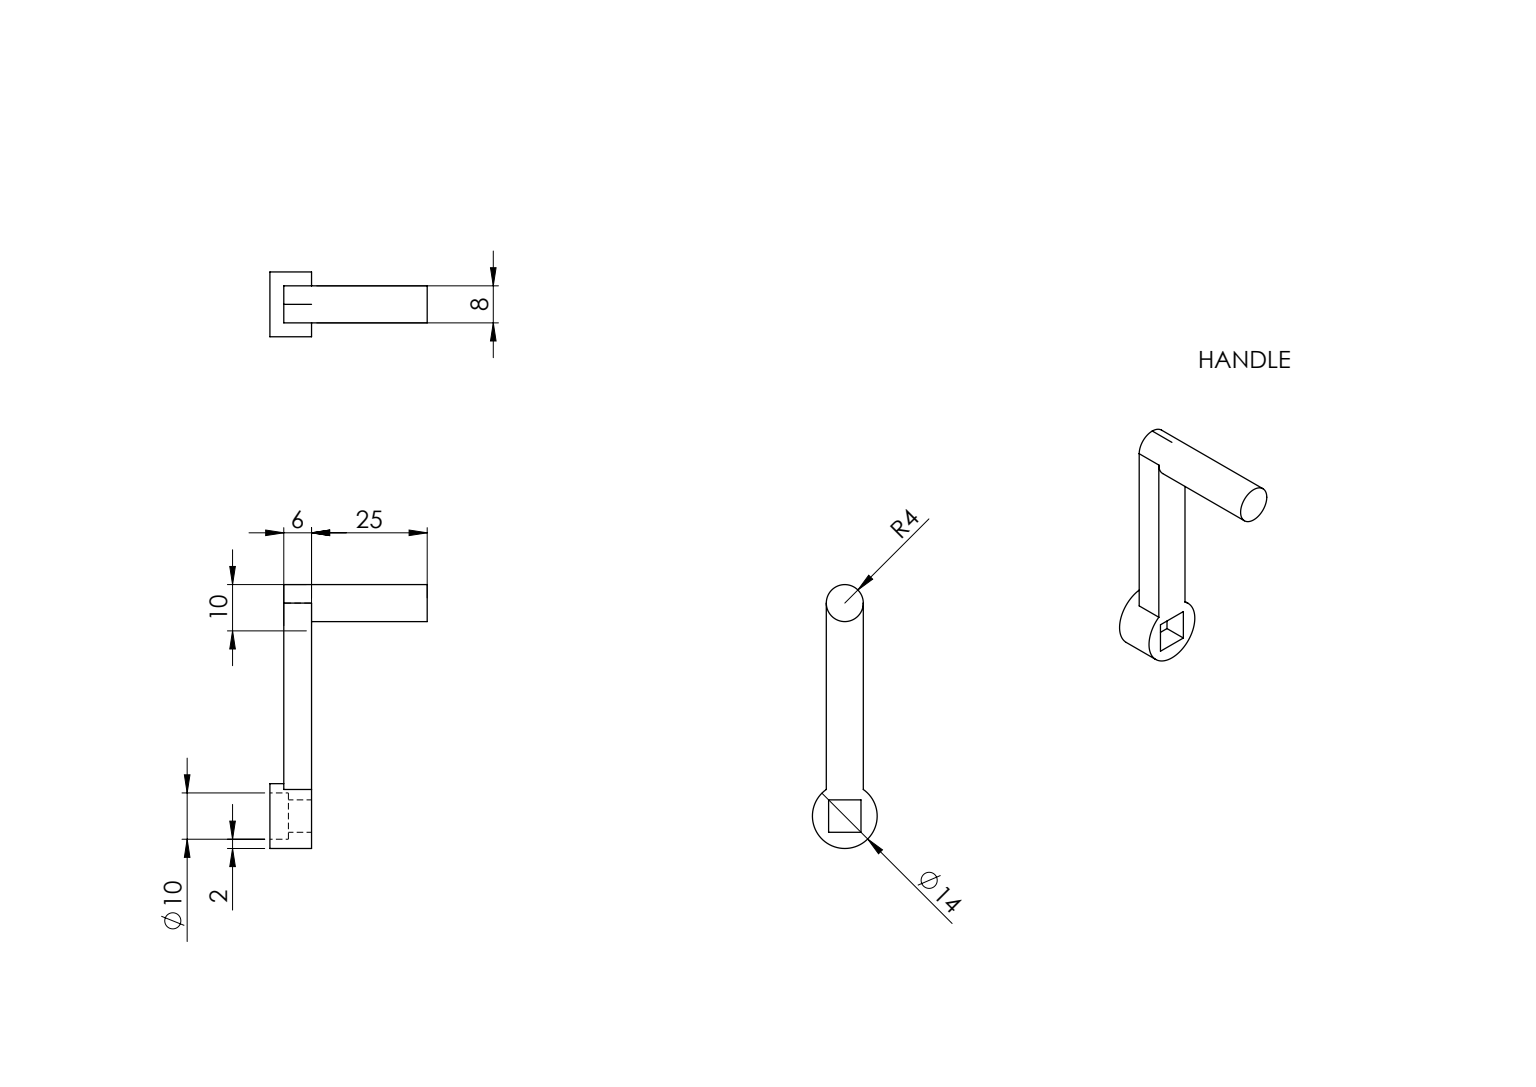
ISO-10303-21;
HEADER;
FILE_DESCRIPTION (('STEP AP214'),
    '1' );
FILE_NAME ('handle.step',
    '2026-10-27T08:02:39',
    ( '' ),
    ( '' ),
    'SwSTEP 2.0',
    'SolidWorks 2026',
    '' );
FILE_SCHEMA (( 'AUTOMOTIVE_DESIGN' ));
ENDSEC;

DATA;
#27=EDGE_LOOP ( 'NONE', ( #3716, #7736, #9091, #8420 ) ) ;
#71=( LENGTH_UNIT ( ) NAMED_UNIT ( * ) SI_UNIT ( .MILLI., .METRE. ) );
#105=LINE ( 'NONE', #3865, #7814 ) ;
#108=EDGE_CURVE ( 'NONE', #8484, #432, #5151, .T. ) ;
#117=DIRECTION ( 'NONE',  ( 0.000000000000000000, 0.000000000000000000, 1.000000000000000000 ) ) ;
#124=DIRECTION ( 'NONE',  ( 0.000000000000000000, 0.000000000000000000, 1.000000000000000000 ) ) ;
#170=VERTEX_POINT ( 'NONE', #7231 ) ;
#212=CARTESIAN_POINT ( 'NONE',  ( 0.000000000000000000, 0.000000000000000000, 0.000000000000000000 ) ) ;
#216=AXIS2_PLACEMENT_3D ( 'NONE', #497, #4306, #3323 ) ;
#249=FACE_OUTER_BOUND ( 'NONE', #9270, .T. ) ;
#265=EDGE_CURVE ( 'NONE', #8484, #2318, #5290, .T. ) ;
#277=CARTESIAN_POINT ( 'NONE',  ( 0.000000000000000000, 46.00000000000001421, -41.99999999999999289 ) ) ;
#311=EDGE_LOOP ( 'NONE', ( #6611, #4902, #12095, #9968, #4063 ) ) ;
#312=LINE ( 'NONE', #2306, #8963 ) ;
#316=CARTESIAN_POINT ( 'NONE',  ( 45.00000000000001421, 50.00000000000000711, -46.00000000000000000 ) ) ;
#333=CARTESIAN_POINT ( 'NONE',  ( 65.79898987322334847, -9.445087446769608850E-17, -41.99999999999998579 ) ) ;
#361=VECTOR ( 'NONE', #839, 1000.000000000000000 ) ;
#362=CARTESIAN_POINT ( 'NONE',  ( 42.00000000000000000, 1.908195823574506293E-17, -41.99999999999998579 ) ) ;
#378=ORIENTED_EDGE ( 'NONE', *, *, #265, .F. ) ;
#413=LINE ( 'NONE', #4060, #11148 ) ;
#432=VERTEX_POINT ( 'NONE', #10181 ) ;
#443=DIRECTION ( 'NONE',  ( 0.000000000000000000, 0.000000000000000000, 1.000000000000000000 ) ) ;
#488=ORIENTED_EDGE ( 'NONE', *, *, #5345, .F. ) ;
#495=EDGE_CURVE ( 'NONE', #1234, #3139, #11361, .T. ) ;
#497=CARTESIAN_POINT ( 'NONE',  ( 45.00000000000001421, 4.770489558936308102E-18, -41.99999999999998579 ) ) ;
#677=CIRCLE ( 'NONE', #7465, 5.000000000000004441 ) ;
#683=AXIS2_PLACEMENT_3D ( 'NONE', #333, #4146, #1473 ) ;
#699=CIRCLE ( 'NONE', #3309, 7.000000000000006217 ) ;
#730=DIRECTION ( 'NONE',  ( 1.000000000000000000, 0.000000000000000000, 0.000000000000000000 ) ) ;
#756=CARTESIAN_POINT ( 'NONE',  ( 65.79898987322334847, -9.445087446769608850E-17, -41.99999999999998579 ) ) ;
#758=AXIS2_PLACEMENT_3D ( 'NONE', #5741, #8694, #117 ) ;
#761=ORIENTED_EDGE ( 'NONE', *, *, #8385, .F. ) ;
#811=VERTEX_POINT ( 'NONE', #6939 ) ;
#839=DIRECTION ( 'NONE',  ( 1.000000000000000000, -4.770489558936236458E-18, 6.855277276495154548E-34 ) ) ;
#858=LINE ( 'NONE', #11064, #11986 ) ;
#871=EDGE_CURVE ( 'NONE', #3139, #7019, #10116, .T. ) ;
#884=EDGE_CURVE ( 'NONE', #5539, #7662, #4798, .T. ) ;
#892=EDGE_LOOP ( 'NONE', ( #2724, #5114, #7799, #6342 ) ) ;
#905=DIRECTION ( 'NONE',  ( -1.000000000000000000, -0.000000000000000000, -0.000000000000000000 ) ) ;
#936=( NAMED_UNIT ( * ) SI_UNIT ( $, .STERADIAN. ) SOLID_ANGLE_UNIT ( ) );
#953=EDGE_CURVE ( 'NONE', #8701, #7793, #8813, .T. ) ;
#960=ORIENTED_EDGE ( 'NONE', *, *, #7258, .T. ) ;
#968=EDGE_CURVE ( 'NONE', #2318, #8881, #10351, .T. ) ;
#999=SURFACE_STYLE_FILL_AREA ( #8572 ) ;
#1040=AXIS2_PLACEMENT_3D ( 'NONE', #277, #8722, #1092 ) ;
#1076=EDGE_CURVE ( 'NONE', #3524, #10474, #105, .T. ) ;
#1092=DIRECTION ( 'NONE',  ( 0.000000000000000000, 0.000000000000000000, -1.000000000000000000 ) ) ;
#1094=VERTEX_POINT ( 'NONE', #10483 ) ;
#1110=DIRECTION ( 'NONE',  ( 1.000000000000000000, 0.000000000000000000, 0.000000000000000000 ) ) ;
#1174=EDGE_CURVE ( 'NONE', #7662, #5539, #10599, .T. ) ;
#1176=DIRECTION ( 'NONE',  ( 1.000000000000000000, 0.000000000000000000, 0.000000000000000000 ) ) ;
#1223=ORIENTED_EDGE ( 'NONE', *, *, #871, .T. ) ;
#1234=VERTEX_POINT ( 'NONE', #9922 ) ;
#1307=DIRECTION ( 'NONE',  ( 1.000000000000000000, -4.770489558936236458E-18, 6.855277276495153692E-34 ) ) ;
#1321=PLANE ( 'NONE',  #8288 ) ;
#1368=CYLINDRICAL_SURFACE ( 'NONE', #11978, 7.000000000000004441 ) ;
#1414=ADVANCED_FACE ( 'NONE', ( #3479 ), #2525, .T. ) ;
#1418=ADVANCED_FACE ( 'NONE', ( #9115 ), #8166, .F. ) ;
#1444=AXIS2_PLACEMENT_3D ( 'NONE', #316, #443, #11744 ) ;
#1473=DIRECTION ( 'NONE',  ( 0.000000000000000000, -1.000000000000000000, 0.000000000000000000 ) ) ;
#1497=EDGE_CURVE ( 'NONE', #8881, #432, #11394, .T. ) ;
#1509=DIRECTION ( 'NONE',  ( -1.000000000000000000, 0.000000000000000000, -0.000000000000000000 ) ) ;
#1515=ORIENTED_EDGE ( 'NONE', *, *, #7216, .T. ) ;
#1552=ADVANCED_FACE ( 'NONE', ( #6730, #2960 ), #4771, .F. ) ;
#1573=DIRECTION ( 'NONE',  ( 0.000000000000000000, 1.000000000000000000, 0.000000000000000000 ) ) ;
#1576=DIRECTION ( 'NONE',  ( 0.000000000000000000, 0.000000000000000000, -1.000000000000000000 ) ) ;
#1590=CARTESIAN_POINT ( 'NONE',  ( 45.00000000000001421, 50.00000000000000711, -38.00000000000000000 ) ) ;
#1622=AXIS2_PLACEMENT_3D ( 'NONE', #4950, #7720, #6772 ) ;
#1645=DIRECTION ( 'NONE',  ( 1.000000000000000000, -0.000000000000000000, 0.000000000000000000 ) ) ;
#1652=FACE_OUTER_BOUND ( 'NONE', #12014, .T. ) ;
#1663=DIRECTION ( 'NONE',  ( 0.000000000000000000, -1.000000000000000000, 0.000000000000000000 ) ) ;
#1696=DIRECTION ( 'NONE',  ( 0.000000000000000000, 0.000000000000000000, 1.000000000000000000 ) ) ;
#1770=AXIS2_PLACEMENT_3D ( 'NONE', #7783, #8594, #8665 ) ;
#1784=SHAPE_DEFINITION_REPRESENTATION ( #10198, #8426 ) ;
#1801=EDGE_CURVE ( 'NONE', #10474, #1992, #3521, .T. ) ;
#1808=VECTOR ( 'NONE', #1573, 1000.000000000000000 ) ;
#1887=( GEOMETRIC_REPRESENTATION_CONTEXT ( 3 ) GLOBAL_UNCERTAINTY_ASSIGNED_CONTEXT ( ( #4523 ) ) GLOBAL_UNIT_ASSIGNED_CONTEXT ( ( #4965, #6678, #5723 ) ) REPRESENTATION_CONTEXT ( 'NONE', 'WORKASPACE' ) );
#1905=VERTEX_POINT ( 'NONE', #4756 ) ;
#1931=CARTESIAN_POINT ( 'NONE',  ( 45.00000000000001421, 46.00000000000001421, -38.00000000000000000 ) ) ;
#1944=SURFACE_STYLE_USAGE ( .BOTH. , #2886 ) ;
#1992=VERTEX_POINT ( 'NONE', #2752 ) ;
#2006=CARTESIAN_POINT ( 'NONE',  ( 76.00000000000000000, 46.00000000000001421, -41.99999999999999289 ) ) ;
#2103=DIRECTION ( 'NONE',  ( -0.000000000000000000, -1.000000000000000000, -0.000000000000000000 ) ) ;
#2106=DIRECTION ( 'NONE',  ( 0.000000000000000000, 0.000000000000000000, -1.000000000000000000 ) ) ;
#2125=( NAMED_UNIT ( * ) PLANE_ANGLE_UNIT ( ) SI_UNIT ( $, .RADIAN. ) );
#2130=DIRECTION ( 'NONE',  ( -1.000000000000000000, 0.000000000000000000, -0.000000000000000000 ) ) ;
#2145=FACE_OUTER_BOUND ( 'NONE', #3394, .T. ) ;
#2163=AXIS2_PLACEMENT_3D ( 'NONE', #7632, #7560, #12296 ) ;
#2184=DIRECTION ( 'NONE',  ( 4.770489558936236458E-18, 1.000000000000000000, 0.000000000000000000 ) ) ;
#2220=ORIENTED_EDGE ( 'NONE', *, *, #9403, .F. ) ;
#2253=EDGE_CURVE ( 'NONE', #1094, #8881, #10596, .T. ) ;
#2293=ORIENTED_EDGE ( 'NONE', *, *, #11296, .T. ) ;
#2306=CARTESIAN_POINT ( 'NONE',  ( 45.00000000000001421, 46.00000000000001421, -46.00000000000000000 ) ) ;
#2318=VERTEX_POINT ( 'NONE', #1931 ) ;
#2319=DIRECTION ( 'NONE',  ( 0.000000000000000000, -1.000000000000000000, 0.000000000000000000 ) ) ;
#2333=EDGE_CURVE ( 'NONE', #8484, #8701, #3056, .T. ) ;
#2385=DIRECTION ( 'NONE',  ( -1.000000000000000000, -0.000000000000000000, -0.000000000000000000 ) ) ;
#2442=ORIENTED_EDGE ( 'NONE', *, *, #9009, .T. ) ;
#2505=EDGE_CURVE ( 'NONE', #1094, #7890, #11958, .T. ) ;
#2508=CARTESIAN_POINT ( 'NONE',  ( 51.00000000000000000, 1.444447458290426890E-31, -41.99999999999998579 ) ) ;
#2525=CYLINDRICAL_SURFACE ( 'NONE', #10013, 7.000000000000004441 ) ;
#2530=ORIENTED_EDGE ( 'NONE', *, *, #6325, .F. ) ;
#2555=CARTESIAN_POINT ( 'NONE',  ( 51.00000000000000000, 5.744562646538031281, -46.00000000000000000 ) ) ;
#2576=EDGE_LOOP ( 'NONE', ( #5137, #9790, #5069, #9510 ) ) ;
#2579=VECTOR ( 'NONE', #6955, 1000.000000000000000 ) ;
#2584=VECTOR ( 'NONE', #5375, 1000.000000000000000 ) ;
#2586=DIRECTION ( 'NONE',  ( 0.000000000000000000, 0.000000000000000000, -1.000000000000000000 ) ) ;
#2603=EDGE_LOOP ( 'NONE', ( #8336, #4066 ) ) ;
#2630=LINE ( 'NONE', #8207, #11415 ) ;
#2671=DIRECTION ( 'NONE',  ( 0.000000000000000000, 0.000000000000000000, -1.000000000000000000 ) ) ;
#2683=PLANE ( 'NONE',  #7968 ) ;
#2694=DIRECTION ( 'NONE',  ( 0.000000000000000000, -1.000000000000000000, 0.000000000000000000 ) ) ;
#2702=ORIENTED_EDGE ( 'NONE', *, *, #953, .F. ) ;
#2724=ORIENTED_EDGE ( 'NONE', *, *, #5874, .F. ) ;
#2752=CARTESIAN_POINT ( 'NONE',  ( 46.00000000000000000, 3.500000000000001332, -45.49999999999998579 ) ) ;
#2762=UNCERTAINTY_MEASURE_WITH_UNIT (LENGTH_MEASURE( 1.000000000000000082E-05 ), #8513, 'distance_accuracy_value', 'NONE');
#2861=ORIENTED_EDGE ( 'NONE', *, *, #7930, .T. ) ;
#2886=SURFACE_SIDE_STYLE ('',( #999 ) ) ;
#2960=FACE_OUTER_BOUND ( 'NONE', #5300, .T. ) ;
#2985=VECTOR ( 'NONE', #12159, 1000.000000000000000 ) ;
#3029=AXIS2_PLACEMENT_3D ( 'NONE', #1590, #2586, #11956 ) ;
#3056=LINE ( 'NONE', #11666, #5020 ) ;
#3059=ADVANCED_FACE ( 'NONE', ( #9861 ), #11652, .T. ) ;
#3121=ADVANCED_FACE ( 'NONE', ( #11137 ), #3649, .F. ) ;
#3136=( NAMED_UNIT ( * ) SI_UNIT ( $, .STERADIAN. ) SOLID_ANGLE_UNIT ( ) );
#3139=VERTEX_POINT ( 'NONE', #12124 ) ;
#3158=DIRECTION ( 'NONE',  ( -0.000000000000000000, 1.000000000000000000, 0.000000000000000000 ) ) ;
#3165=ORIENTED_EDGE ( 'NONE', *, *, #8385, .T. ) ;
#3177=CARTESIAN_POINT ( 'NONE',  ( 51.00000000000000000, 3.500000000000001332, -38.49999999999998579 ) ) ;
#3185=VECTOR ( 'NONE', #11275, 1000.000000000000000 ) ;
#3212=DIRECTION ( 'NONE',  ( 0.000000000000000000, -0.000000000000000000, -1.000000000000000000 ) ) ;
#3309=AXIS2_PLACEMENT_3D ( 'NONE', #2508, #6330, #1696 ) ;
#3323=DIRECTION ( 'NONE',  ( 0.000000000000000000, 2.664535259100374514E-15, 1.000000000000000000 ) ) ;
#3344=ORIENTED_EDGE ( 'NONE', *, *, #6728, .F. ) ;
#3349=CARTESIAN_POINT ( 'NONE',  ( 65.79898987322334847, 7.000000000000004441, -41.99999999999998579 ) ) ;
#3394=EDGE_LOOP ( 'NONE', ( #10298, #8483, #1515, #2702 ) ) ;
#3408=DIRECTION ( 'NONE',  ( -1.000000000000000000, 4.770489558936236458E-18, -6.855277276495154548E-34 ) ) ;
#3416=ADVANCED_FACE ( 'NONE', ( #9894 ), #5953, .F. ) ;
#3423=AXIS2_PLACEMENT_3D ( 'NONE', #7291, #1110, #4922 ) ;
#3432=ORIENTED_EDGE ( 'NONE', *, *, #11724, .T. ) ;
#3451=ORIENTED_EDGE ( 'NONE', *, *, #2333, .T. ) ;
#3452=FACE_OUTER_BOUND ( 'NONE', #892, .T. ) ;
#3479=FACE_OUTER_BOUND ( 'NONE', #9340, .T. ) ;
#3482=ORIENTED_EDGE ( 'NONE', *, *, #6191, .T. ) ;
#3499=AXIS2_PLACEMENT_3D ( 'NONE', #362, #1307, #2184 ) ;
#3521=LINE ( 'NONE', #4324, #10151 ) ;
#3524=VERTEX_POINT ( 'NONE', #6903 ) ;
#3526=DIRECTION ( 'NONE',  ( 0.000000000000000000, 0.000000000000000000, 1.000000000000000000 ) ) ;
#3527=VERTEX_POINT ( 'NONE', #10704 ) ;
#3538=ORIENTED_EDGE ( 'NONE', *, *, #5874, .T. ) ;
#3545=DIRECTION ( 'NONE',  ( -1.000000000000000000, 4.770489558936236458E-18, -6.855277276495154548E-34 ) ) ;
#3570=ORIENTED_EDGE ( 'NONE', *, *, #8614, .F. ) ;
#3586=DIRECTION ( 'NONE',  ( -1.000000000000000000, 0.000000000000000000, 0.000000000000000000 ) ) ;
#3588=ORIENTED_EDGE ( 'NONE', *, *, #265, .T. ) ;
#3632=ORIENTED_EDGE ( 'NONE', *, *, #953, .T. ) ;
#3649=PLANE ( 'NONE',  #7440 ) ;
#3673=DIRECTION ( 'NONE',  ( -1.000000000000000000, 4.770489558936236458E-18, -6.855277276495154548E-34 ) ) ;
#3678=CARTESIAN_POINT ( 'NONE',  ( 76.00000000000000000, 46.00000000000001421, -41.99999999999999289 ) ) ;
#3716=ORIENTED_EDGE ( 'NONE', *, *, #1076, .F. ) ;
#3819=FILL_AREA_STYLE_COLOUR ( '', #6637 ) ;
#3865=CARTESIAN_POINT ( 'NONE',  ( 51.00000000000000000, 3.500000000000001332, -45.49999999999998579 ) ) ;
#3934=APPLICATION_CONTEXT ( 'automotive_design' ) ;
#3941=CARTESIAN_POINT ( 'NONE',  ( 42.00000000000000000, 1.908195823574506293E-17, -41.99999999999998579 ) ) ;
#4025=ADVANCED_FACE ( 'NONE', ( #3452 ), #4311, .T. ) ;
#4033=VERTEX_POINT ( 'NONE', #2555 ) ;
#4035=DIRECTION ( 'NONE',  ( 0.000000000000000000, 0.000000000000000000, 1.000000000000000000 ) ) ;
#4060=CARTESIAN_POINT ( 'NONE',  ( 0.000000000000000000, 46.00000000000001421, -46.00000000000000000 ) ) ;
#4063=ORIENTED_EDGE ( 'NONE', *, *, #968, .F. ) ;
#4066=ORIENTED_EDGE ( 'NONE', *, *, #6164, .F. ) ;
#4135=LINE ( 'NONE', #7903, #2579 ) ;
#4146=DIRECTION ( 'NONE',  ( -1.000000000000000000, 4.770489558936235687E-18, -6.855277276495154548E-34 ) ) ;
#4153=DIRECTION ( 'NONE',  ( 0.000000000000000000, 0.000000000000000000, -1.000000000000000000 ) ) ;
#4207=FACE_OUTER_BOUND ( 'NONE', #9244, .T. ) ;
#4224=ORIENTED_EDGE ( 'NONE', *, *, #7009, .F. ) ;
#4226=ORIENTED_EDGE ( 'NONE', *, *, #5142, .T. ) ;
#4234=DIRECTION ( 'NONE',  ( 1.000000000000000000, 0.000000000000000000, 0.000000000000000000 ) ) ;
#4252=DIRECTION ( 'NONE',  ( -1.000000000000000000, 4.770489558936235687E-18, -6.855277276495154548E-34 ) ) ;
#4258=DIRECTION ( 'NONE',  ( 0.000000000000000000, 0.000000000000000000, -1.000000000000000000 ) ) ;
#4261=ORIENTED_EDGE ( 'NONE', *, *, #7009, .T. ) ;
#4292=LINE ( 'NONE', #11906, #11931 ) ;
#4306=DIRECTION ( 'NONE',  ( 1.000000000000000000, -0.000000000000000000, -0.000000000000000000 ) ) ;
#4311=PLANE ( 'NONE',  #10450 ) ;
#4324=CARTESIAN_POINT ( 'NONE',  ( 70.79898987322334847, 3.500000000000001332, -45.49999999999998579 ) ) ;
#4334=ADVANCED_FACE ( 'NONE', ( #249 ), #6068, .T. ) ;
#4335=EDGE_CURVE ( 'NONE', #7138, #5192, #677, .T. ) ;
#4351=ORIENTED_EDGE ( 'NONE', *, *, #5142, .F. ) ;
#4358=ADVANCED_BREP_SHAPE_REPRESENTATION ( '', ( #4548, #6056 ), #7232 ) ;
#4390=FACE_OUTER_BOUND ( 'NONE', #10296, .T. ) ;
#4419=VECTOR ( 'NONE', #7810, 1000.000000000000000 ) ;
#4443=ORIENTED_EDGE ( 'NONE', *, *, #1497, .T. ) ;
#4455=DIRECTION ( 'NONE',  ( 0.000000000000000000, 0.000000000000000000, 1.000000000000000000 ) ) ;
#4466=ORIENTED_EDGE ( 'NONE', *, *, #968, .T. ) ;
#4509=ORIENTED_EDGE ( 'NONE', *, *, #6191, .F. ) ;
#4523=UNCERTAINTY_MEASURE_WITH_UNIT (LENGTH_MEASURE( 1.000000000000000082E-05 ), #4965, 'distance_accuracy_value', 'NONE');
#4548=MANIFOLD_SOLID_BREP ( 'Boss-Extrude3', #6364 ) ;
#4583=VECTOR ( 'NONE', #2103, 1000.000000000000000 ) ;
#4602=LINE ( 'NONE', #6682, #6605 ) ;
#4625=ADVANCED_FACE ( 'NONE', ( #4207 ), #7043, .F. ) ;
#4629=EDGE_CURVE ( 'NONE', #3527, #4033, #7864, .T. ) ;
#4655=ORIENTED_EDGE ( 'NONE', *, *, #6727, .T. ) ;
#4677=DIRECTION ( 'NONE',  ( 0.000000000000000000, 0.000000000000000000, -1.000000000000000000 ) ) ;
#4692=ORIENTED_EDGE ( 'NONE', *, *, #2253, .F. ) ;
#4707=PLANE ( 'NONE',  #6031 ) ;
#4756=CARTESIAN_POINT ( 'NONE',  ( 45.00000000000001421, 5.744562646538025952, -46.00000000000000000 ) ) ;
#4771=PLANE ( 'NONE',  #1770 ) ;
#4792=CARTESIAN_POINT ( 'NONE',  ( 51.00000000000000000, -3.499999999999998668, -38.49999999999998579 ) ) ;
#4798=CIRCLE ( 'NONE', #11770, 5.000000000000004441 ) ;
#4818=CARTESIAN_POINT ( 'NONE',  ( 51.00000000000000000, -3.499999999999998668, -45.49999999999998579 ) ) ;
#4821=STYLED_ITEM ( 'NONE', ( #5747 ), #4358 ) ;
#4900=VECTOR ( 'NONE', #11734, 1000.000000000000000 ) ;
#4902=ORIENTED_EDGE ( 'NONE', *, *, #10762, .T. ) ;
#4913=ORIENTED_EDGE ( 'NONE', *, *, #2505, .F. ) ;
#4922=DIRECTION ( 'NONE',  ( 0.000000000000000000, 0.000000000000000000, -1.000000000000000000 ) ) ;
#4950=CARTESIAN_POINT ( 'NONE',  ( 42.00000000000000000, 1.908195823574506293E-17, -41.99999999999998579 ) ) ;
#4958=ADVANCED_FACE ( 'NONE', ( #11822 ), #1321, .T. ) ;
#4965=( LENGTH_UNIT ( ) NAMED_UNIT ( * ) SI_UNIT ( .MILLI., .METRE. ) );
#5020=VECTOR ( 'NONE', #6928, 1000.000000000000000 ) ;
#5025=CYLINDRICAL_SURFACE ( 'NONE', #1040, 4.000000000000003553 ) ;
#5069=ORIENTED_EDGE ( 'NONE', *, *, #871, .F. ) ;
#5114=ORIENTED_EDGE ( 'NONE', *, *, #495, .T. ) ;
#5137=ORIENTED_EDGE ( 'NONE', *, *, #7930, .F. ) ;
#5138=DIRECTION ( 'NONE',  ( 0.000000000000000000, 3.552713678800500140E-15, 1.000000000000000000 ) ) ;
#5142=EDGE_CURVE ( 'NONE', #9147, #432, #699, .T. ) ;
#5151=LINE ( 'NONE', #9920, #4583 ) ;
#5179=EDGE_LOOP ( 'NONE', ( #3538, #7191, #5649, #2861 ) ) ;
#5181=VECTOR ( 'NONE', #10482, 1000.000000000000000 ) ;
#5186=CARTESIAN_POINT ( 'NONE',  ( 65.79898987322334847, -9.445087446769608850E-17, -41.99999999999998579 ) ) ;
#5192=VERTEX_POINT ( 'NONE', #7336 ) ;
#5198=EDGE_LOOP ( 'NONE', ( #10888, #4261 ) ) ;
#5206=APPLICATION_CONTEXT ( 'automotive_design' ) ;
#5225=AXIS2_PLACEMENT_3D ( 'NONE', #11646, #8962, #5138 ) ;
#5290=LINE ( 'NONE', #9294, #3185 ) ;
#5292=CARTESIAN_POINT ( 'NONE',  ( 65.79898987322334847, -9.445087446769608850E-17, -41.99999999999998579 ) ) ;
#5300=EDGE_LOOP ( 'NONE', ( #9607, #9219 ) ) ;
#5345=EDGE_CURVE ( 'NONE', #10474, #9620, #10449, .T. ) ;
#5353=DIRECTION ( 'NONE',  ( 1.000000000000000000, -4.770489558936235687E-18, 6.855277276495153692E-34 ) ) ;
#5371=ADVANCED_FACE ( 'NONE', ( #10812, #7759 ), #8758, .F. ) ;
#5375=DIRECTION ( 'NONE',  ( -1.000000000000000000, -0.000000000000000000, -0.000000000000000000 ) ) ;
#5399=CYLINDRICAL_SURFACE ( 'NONE', #9177, 5.000000000000004441 ) ;
#5438=AXIS2_PLACEMENT_3D ( 'NONE', #8489, #12220, #2671 ) ;
#5461=CARTESIAN_POINT ( 'NONE',  ( 46.00000000000000000, -3.499999999999998668, -45.49999999999998579 ) ) ;
#5539=VERTEX_POINT ( 'NONE', #8262 ) ;
#5549=LINE ( 'NONE', #8363, #2985 ) ;
#5550=ORIENTED_EDGE ( 'NONE', *, *, #4629, .F. ) ;
#5560=ORIENTED_EDGE ( 'NONE', *, *, #6727, .F. ) ;
#5591=ORIENTED_EDGE ( 'NONE', *, *, #108, .F. ) ;
#5598=VECTOR ( 'NONE', #4677, 1000.000000000000000 ) ;
#5649=ORIENTED_EDGE ( 'NONE', *, *, #5345, .T. ) ;
#5723=( NAMED_UNIT ( * ) SI_UNIT ( $, .STERADIAN. ) SOLID_ANGLE_UNIT ( ) );
#5733=CARTESIAN_POINT ( 'NONE',  ( 51.00000000000000000, -7.000000000000007994, -41.99999999999998579 ) ) ;
#5741=CARTESIAN_POINT ( 'NONE',  ( 51.00000000000000000, 1.444447458290426890E-31, -41.99999999999998579 ) ) ;
#5747=PRESENTATION_STYLE_ASSIGNMENT (( #1944 ) ) ;
#5874=EDGE_CURVE ( 'NONE', #1234, #3524, #7881, .T. ) ;
#5887=ORIENTED_EDGE ( 'NONE', *, *, #884, .T. ) ;
#5935=ORIENTED_EDGE ( 'NONE', *, *, #6164, .T. ) ;
#5948=DIRECTION ( 'NONE',  ( 0.000000000000000000, 0.000000000000000000, -1.000000000000000000 ) ) ;
#5953=PLANE ( 'NONE',  #1444 ) ;
#5966=CIRCLE ( 'NONE', #758, 7.000000000000006217 ) ;
#6012=CARTESIAN_POINT ( 'NONE',  ( 45.00000000000001421, 5.744562646538041051, -38.00000000000000000 ) ) ;
#6015=VECTOR ( 'NONE', #3408, 1000.000000000000000 ) ;
#6027=PRODUCT_DEFINITION_CONTEXT ( 'detailed design', #3934, 'design' ) ;
#6028=VERTEX_POINT ( 'NONE', #8302 ) ;
#6031=AXIS2_PLACEMENT_3D ( 'NONE', #12259, #3586, #3526 ) ;
#6056=AXIS2_PLACEMENT_3D ( 'NONE', #212, #4035, #8864 ) ;
#6068=PLANE ( 'NONE',  #9466 ) ;
#6077=FACE_OUTER_BOUND ( 'NONE', #10669, .T. ) ;
#6164=EDGE_CURVE ( 'NONE', #7890, #170, #6831, .T. ) ;
#6182=ORIENTED_EDGE ( 'NONE', *, *, #6452, .T. ) ;
#6191=EDGE_CURVE ( 'NONE', #9147, #170, #4602, .T. ) ;
#6278=STYLED_ITEM('',(#12391),#4548);
#6325=EDGE_CURVE ( 'NONE', #1905, #1094, #6838, .T. ) ;
#6330=DIRECTION ( 'NONE',  ( -1.000000000000000000, 0.000000000000000000, 0.000000000000000000 ) ) ;
#6342=ORIENTED_EDGE ( 'NONE', *, *, #7843, .F. ) ;
#6347=DIRECTION ( 'NONE',  ( -1.000000000000000000, 4.770489558936235687E-18, -6.855277276495154548E-34 ) ) ;
#6364=CLOSED_SHELL ( 'NONE', ( #11110, #4625, #8884, #1414, #5371, #7538, #1552, #4025, #3059, #4334, #4958, #11135, #3416, #3121, #1418, #9601, #7076 ) ) ;
#6390=EDGE_CURVE ( 'NONE', #6028, #3139, #2630, .T. ) ;
#6446=CARTESIAN_POINT ( 'NONE',  ( 70.79898987322334847, -3.499999999999998668, -38.49999999999998579 ) ) ;
#6452=EDGE_CURVE ( 'NONE', #1992, #6028, #11131, .T. ) ;
#6517=LINE ( 'NONE', #5461, #1808 ) ;
#6605=VECTOR ( 'NONE', #3673, 1000.000000000000000 ) ;
#6611=ORIENTED_EDGE ( 'NONE', *, *, #6728, .T. ) ;
#6616=AXIS2_PLACEMENT_3D ( 'NONE', #10964, #6978, #4153 ) ;
#6637=COLOUR_RGB ( '',0.8941176470588234615, 0.8941176470588234615, 0.8941176470588234615 ) ;
#6670=LINE ( 'NONE', #9593, #9392 ) ;
#6678=( NAMED_UNIT ( * ) PLANE_ANGLE_UNIT ( ) SI_UNIT ( $, .RADIAN. ) );
#6682=CARTESIAN_POINT ( 'NONE',  ( 65.79898987322334847, -7.000000000000004441, -41.99999999999998579 ) ) ;
#6726=ORIENTED_EDGE ( 'NONE', *, *, #2505, .T. ) ;
#6727=EDGE_CURVE ( 'NONE', #811, #3527, #312, .T. ) ;
#6728=EDGE_CURVE ( 'NONE', #2318, #811, #7795, .T. ) ;
#6729=DIRECTION ( 'NONE',  ( -1.000000000000000000, 4.770489558936236458E-18, -6.855277276495154548E-34 ) ) ;
#6730=FACE_BOUND ( 'NONE', #6809, .T. ) ;
#6772=DIRECTION ( 'NONE',  ( 0.000000000000000000, 0.000000000000000000, -1.000000000000000000 ) ) ;
#6809=EDGE_LOOP ( 'NONE', ( #9106, #1223, #6929, #6182 ) ) ;
#6831=CIRCLE ( 'NONE', #5438, 7.000000000000006217 ) ;
#6838=CIRCLE ( 'NONE', #5225, 7.000000000000006217 ) ;
#6846=CARTESIAN_POINT ( 'NONE',  ( 42.00000000000000000, 7.000000000000004441, -41.99999999999998579 ) ) ;
#6903=CARTESIAN_POINT ( 'NONE',  ( 51.00000000000000000, 3.500000000000001332, -38.49999999999998579 ) ) ;
#6915=CARTESIAN_POINT ( 'NONE',  ( 70.79898987322334847, -3.499999999999998668, -38.49999999999998579 ) ) ;
#6928=DIRECTION ( 'NONE',  ( 1.000000000000000000, 0.000000000000000000, 0.000000000000000000 ) ) ;
#6929=ORIENTED_EDGE ( 'NONE', *, *, #8614, .T. ) ;
#6939=CARTESIAN_POINT ( 'NONE',  ( 45.00000000000001421, 46.00000000000001421, -46.00000000000000000 ) ) ;
#6955=DIRECTION ( 'NONE',  ( -1.000000000000000000, -0.000000000000000000, -0.000000000000000000 ) ) ;
#6978=DIRECTION ( 'NONE',  ( 1.000000000000000000, 0.000000000000000000, 0.000000000000000000 ) ) ;
#7009=EDGE_CURVE ( 'NONE', #5192, #7138, #10344, .T. ) ;
#7019=VERTEX_POINT ( 'NONE', #10494 ) ;
#7034=EDGE_CURVE ( 'NONE', #4033, #9147, #5966, .T. ) ;
#7043=CYLINDRICAL_SURFACE ( 'NONE', #683, 5.000000000000004441 ) ;
#7076=ADVANCED_FACE ( 'NONE', ( #9375 ), #2683, .T. ) ;
#7116=ORIENTED_EDGE ( 'NONE', *, *, #10580, .F. ) ;
#7130=DIRECTION ( 'NONE',  ( 1.000000000000000000, -0.000000000000000000, -0.000000000000000000 ) ) ;
#7138=VERTEX_POINT ( 'NONE', #7812 ) ;
#7191=ORIENTED_EDGE ( 'NONE', *, *, #1076, .T. ) ;
#7203=CARTESIAN_POINT ( 'NONE',  ( 70.79898987322334847, 3.500000000000001332, -38.49999999999998579 ) ) ;
#7216=EDGE_CURVE ( 'NONE', #3527, #7793, #413, .T. ) ;
#7231=CARTESIAN_POINT ( 'NONE',  ( 42.00000000000000000, -7.000000000000004441, -41.99999999999998579 ) ) ;
#7232=( GEOMETRIC_REPRESENTATION_CONTEXT ( 3 ) GLOBAL_UNCERTAINTY_ASSIGNED_CONTEXT ( ( #2762 ) ) GLOBAL_UNIT_ASSIGNED_CONTEXT ( ( #8513, #7707, #936 ) ) REPRESENTATION_CONTEXT ( 'NONE', 'WORKASPACE' ) );
#7258=EDGE_CURVE ( 'NONE', #5539, #7138, #4292, .T. ) ;
#7291=CARTESIAN_POINT ( 'NONE',  ( 0.000000000000000000, 46.00000000000001421, -41.99999999999999289 ) ) ;
#7316=CARTESIAN_POINT ( 'NONE',  ( 46.00000000000000000, -3.499999999999998668, -38.49999999999998579 ) ) ;
#7336=CARTESIAN_POINT ( 'NONE',  ( 42.00000000000000000, 5.000000000000004441, -41.99999999999998579 ) ) ;
#7365=CARTESIAN_POINT ( 'NONE',  ( 46.00000000000000000, 1.444447458290426890E-31, -41.99999999999998579 ) ) ;
#7428=( GEOMETRIC_REPRESENTATION_CONTEXT ( 3 ) GLOBAL_UNCERTAINTY_ASSIGNED_CONTEXT ( ( #9406 ) ) GLOBAL_UNIT_ASSIGNED_CONTEXT ( ( #71, #2125, #3136 ) ) REPRESENTATION_CONTEXT ( 'NONE', 'WORKASPACE' ) );
#7432=VECTOR ( 'NONE', #4455, 1000.000000000000000 ) ;
#7434=DIRECTION ( 'NONE',  ( 1.000000000000000000, 0.000000000000000000, 0.000000000000000000 ) ) ;
#7440=AXIS2_PLACEMENT_3D ( 'NONE', #10144, #1645, #1576 ) ;
#7465=AXIS2_PLACEMENT_3D ( 'NONE', #3941, #5353, #9305 ) ;
#7497=DIRECTION ( 'NONE',  ( 0.000000000000000000, 0.000000000000000000, -1.000000000000000000 ) ) ;
#7538=ADVANCED_FACE ( 'NONE', ( #12126 ), #5399, .F. ) ;
#7550=DIRECTION ( 'NONE',  ( -1.000000000000000000, 4.770489558936236458E-18, -6.855277276495154548E-34 ) ) ;
#7554=PRODUCT_DEFINITION ( 'UNKNOWN', '', #9649, #6027 ) ;
#7560=DIRECTION ( 'NONE',  ( 1.000000000000000000, -4.770489558936235687E-18, 6.855277276495153692E-34 ) ) ;
#7632=CARTESIAN_POINT ( 'NONE',  ( 42.00000000000000000, 1.908195823574506293E-17, -41.99999999999998579 ) ) ;
#7662=VERTEX_POINT ( 'NONE', #11384 ) ;
#7707=( NAMED_UNIT ( * ) PLANE_ANGLE_UNIT ( ) SI_UNIT ( $, .RADIAN. ) );
#7720=DIRECTION ( 'NONE',  ( 1.000000000000000000, -4.770489558936235687E-18, 6.855277276495153692E-34 ) ) ;
#7736=ORIENTED_EDGE ( 'NONE', *, *, #7843, .T. ) ;
#7739=LINE ( 'NONE', #4792, #5181 ) ;
#7759=FACE_BOUND ( 'NONE', #5198, .T. ) ;
#7783=CARTESIAN_POINT ( 'NONE',  ( 46.00000000000000000, 1.444447458290426890E-31, -41.99999999999998579 ) ) ;
#7793=VERTEX_POINT ( 'NONE', #10886 ) ;
#7795=CIRCLE ( 'NONE', #11141, 4.000000000000003553 ) ;
#7799=ORIENTED_EDGE ( 'NONE', *, *, #6390, .F. ) ;
#7810=DIRECTION ( 'NONE',  ( 0.000000000000000000, 1.000000000000000000, 0.000000000000000000 ) ) ;
#7812=CARTESIAN_POINT ( 'NONE',  ( 42.00000000000000000, -5.000000000000004441, -41.99999999999998579 ) ) ;
#7814=VECTOR ( 'NONE', #2106, 1000.000000000000000 ) ;
#7830=ORIENTED_EDGE ( 'NONE', *, *, #7034, .T. ) ;
#7832=MECHANICAL_DESIGN_GEOMETRIC_PRESENTATION_REPRESENTATION('',(#4821),#7428);
#7843=EDGE_CURVE ( 'NONE', #3524, #6028, #4135, .T. ) ;
#7864=LINE ( 'NONE', #11657, #11457 ) ;
#7881=LINE ( 'NONE', #3177, #4419 ) ;
#7890=VERTEX_POINT ( 'NONE', #6846 ) ;
#7903=CARTESIAN_POINT ( 'NONE',  ( 70.79898987322334847, 3.500000000000001332, -38.49999999999998579 ) ) ;
#7930=EDGE_CURVE ( 'NONE', #9620, #1234, #7739, .T. ) ;
#7955=ORIENTED_EDGE ( 'NONE', *, *, #1801, .T. ) ;
#7960=CARTESIAN_POINT ( 'NONE',  ( 70.79898987322334847, 3.500000000000001332, -45.49999999999998579 ) ) ;
#7968=AXIS2_PLACEMENT_3D ( 'NONE', #10304, #9506, #9854 ) ;
#7999=DIRECTION ( 'NONE',  ( 0.000000000000000000, 0.000000000000000000, -1.000000000000000000 ) ) ;
#8051=DIRECTION ( 'NONE',  ( -0.000000000000000000, -1.000000000000000000, -0.000000000000000000 ) ) ;
#8166=PLANE ( 'NONE',  #3029 ) ;
#8207=CARTESIAN_POINT ( 'NONE',  ( 46.00000000000000000, 3.500000000000001332, -38.49999999999998579 ) ) ;
#8210=VECTOR ( 'NONE', #8308, 1000.000000000000000 ) ;
#8262=CARTESIAN_POINT ( 'NONE',  ( 46.00000000000000000, -5.000000000000004441, -41.99999999999998579 ) ) ;
#8288=AXIS2_PLACEMENT_3D ( 'NONE', #7960, #2319, #3212 ) ;
#8302=CARTESIAN_POINT ( 'NONE',  ( 46.00000000000000000, 3.500000000000001332, -38.49999999999998579 ) ) ;
#8308=DIRECTION ( 'NONE',  ( -0.000000000000000000, -1.000000000000000000, -0.000000000000000000 ) ) ;
#8336=ORIENTED_EDGE ( 'NONE', *, *, #11296, .F. ) ;
#8363=CARTESIAN_POINT ( 'NONE',  ( 45.00000000000001421, 50.00000000000000711, -46.00000000000000000 ) ) ;
#8385=EDGE_CURVE ( 'NONE', #7662, #5192, #6670, .T. ) ;
#8420=ORIENTED_EDGE ( 'NONE', *, *, #1801, .F. ) ;
#8426=SHAPE_REPRESENTATION ( 'handle', ( #6056 ), #7232 ) ;
#8452=ORIENTED_EDGE ( 'NONE', *, *, #1497, .F. ) ;
#8483=ORIENTED_EDGE ( 'NONE', *, *, #10580, .T. ) ;
#8484=VERTEX_POINT ( 'NONE', #9725 ) ;
#8489=CARTESIAN_POINT ( 'NONE',  ( 42.00000000000000000, 1.908195823574506293E-17, -41.99999999999998579 ) ) ;
#8513=( LENGTH_UNIT ( ) NAMED_UNIT ( * ) SI_UNIT ( .MILLI., .METRE. ) );
#8572=FILL_AREA_STYLE ('',( #3819 ) ) ;
#8594=DIRECTION ( 'NONE',  ( 1.000000000000000000, 0.000000000000000000, 0.000000000000000000 ) ) ;
#8614=EDGE_CURVE ( 'NONE', #7019, #1992, #6517, .T. ) ;
#8665=DIRECTION ( 'NONE',  ( 0.000000000000000000, 0.000000000000000000, -1.000000000000000000 ) ) ;
#8682=MECHANICAL_DESIGN_GEOMETRIC_PRESENTATION_REPRESENTATION('',(#6278),#1887);
#8694=DIRECTION ( 'NONE',  ( -1.000000000000000000, 0.000000000000000000, 0.000000000000000000 ) ) ;
#8701=VERTEX_POINT ( 'NONE', #8764 ) ;
#8722=DIRECTION ( 'NONE',  ( 1.000000000000000000, 0.000000000000000000, 0.000000000000000000 ) ) ;
#8758=PLANE ( 'NONE',  #3499 ) ;
#8759=ORIENTED_EDGE ( 'NONE', *, *, #7258, .F. ) ;
#8764=CARTESIAN_POINT ( 'NONE',  ( 76.00000000000000000, 46.00000000000001421, -37.99999999999999289 ) ) ;
#8807=EDGE_LOOP ( 'NONE', ( #761, #11088, #960, #4224 ) ) ;
#8813=CIRCLE ( 'NONE', #9214, 4.000000000000003553 ) ;
#8822=CARTESIAN_POINT ( 'NONE',  ( 70.79898987322334847, -3.499999999999998668, -45.49999999999998579 ) ) ;
#8833=CIRCLE ( 'NONE', #11013, 4.000000000000003553 ) ;
#8864=DIRECTION ( 'NONE',  ( 1.000000000000000000, 0.000000000000000000, 0.000000000000000000 ) ) ;
#8881=VERTEX_POINT ( 'NONE', #6012 ) ;
#8884=ADVANCED_FACE ( 'NONE', ( #6077 ), #1368, .T. ) ;
#8962=DIRECTION ( 'NONE',  ( 1.000000000000000000, -0.000000000000000000, -0.000000000000000000 ) ) ;
#8963=VECTOR ( 'NONE', #7130, 1000.000000000000000 ) ;
#8986=EDGE_LOOP ( 'NONE', ( #11961, #4655, #12174, #2442 ) ) ;
#9003=CARTESIAN_POINT ( 'NONE',  ( 51.00000000000000000, 46.00000000000001421, -41.99999999999999289 ) ) ;
#9009=EDGE_CURVE ( 'NONE', #4033, #1905, #858, .T. ) ;
#9091=ORIENTED_EDGE ( 'NONE', *, *, #6452, .F. ) ;
#9106=ORIENTED_EDGE ( 'NONE', *, *, #6390, .T. ) ;
#9115=FACE_OUTER_BOUND ( 'NONE', #9863, .T. ) ;
#9118=ORIENTED_EDGE ( 'NONE', *, *, #9009, .F. ) ;
#9147=VERTEX_POINT ( 'NONE', #5733 ) ;
#9177=AXIS2_PLACEMENT_3D ( 'NONE', #756, #11943, #9287 ) ;
#9214=AXIS2_PLACEMENT_3D ( 'NONE', #3678, #730, #7497 ) ;
#9219=ORIENTED_EDGE ( 'NONE', *, *, #1174, .F. ) ;
#9244=EDGE_LOOP ( 'NONE', ( #5887, #3165, #9827, #8759 ) ) ;
#9270=EDGE_LOOP ( 'NONE', ( #488, #7955, #3570, #2220 ) ) ;
#9287=DIRECTION ( 'NONE',  ( 0.000000000000000000, -1.000000000000000000, 0.000000000000000000 ) ) ;
#9294=CARTESIAN_POINT ( 'NONE',  ( 45.00000000000001421, 46.00000000000001421, -38.00000000000000000 ) ) ;
#9305=DIRECTION ( 'NONE',  ( 0.000000000000000000, 1.000000000000000000, 0.000000000000000000 ) ) ;
#9340=EDGE_LOOP ( 'NONE', ( #4913, #2530, #9118, #7830, #3482, #2293 ) ) ;
#9375=FACE_OUTER_BOUND ( 'NONE', #11074, .T. ) ;
#9392=VECTOR ( 'NONE', #6729, 1000.000000000000000 ) ;
#9403=EDGE_CURVE ( 'NONE', #9620, #7019, #11217, .T. ) ;
#9406=UNCERTAINTY_MEASURE_WITH_UNIT (LENGTH_MEASURE( 1.000000000000000082E-05 ), #71, 'distance_accuracy_value', 'NONE');
#9410=CARTESIAN_POINT ( 'NONE',  ( 65.79898987322334847, 5.744562646538041051, -38.00000000000000000 ) ) ;
#9466=AXIS2_PLACEMENT_3D ( 'NONE', #8822, #124, #9885 ) ;
#9506=DIRECTION ( 'NONE',  ( 1.000000000000000000, 0.000000000000000000, 0.000000000000000000 ) ) ;
#9510=ORIENTED_EDGE ( 'NONE', *, *, #495, .F. ) ;
#9593=CARTESIAN_POINT ( 'NONE',  ( 65.79898987322334847, 5.000000000000004441, -41.99999999999998579 ) ) ;
#9601=ADVANCED_FACE ( 'NONE', ( #2145 ), #5025, .T. ) ;
#9607=ORIENTED_EDGE ( 'NONE', *, *, #884, .F. ) ;
#9620=VERTEX_POINT ( 'NONE', #11396 ) ;
#9649=PRODUCT_DEFINITION_FORMATION_WITH_SPECIFIED_SOURCE ( 'ANY', '', #12085, .NOT_KNOWN. ) ;
#9711=CARTESIAN_POINT ( 'NONE',  ( 45.00000000000001421, 46.00000000000001421, -41.99999999999999289 ) ) ;
#9725=CARTESIAN_POINT ( 'NONE',  ( 51.00000000000000711, 46.00000000000001421, -38.00000000000000000 ) ) ;
#9790=ORIENTED_EDGE ( 'NONE', *, *, #9403, .T. ) ;
#9827=ORIENTED_EDGE ( 'NONE', *, *, #4335, .F. ) ;
#9854=DIRECTION ( 'NONE',  ( 0.000000000000000000, 0.000000000000000000, -1.000000000000000000 ) ) ;
#9861=FACE_OUTER_BOUND ( 'NONE', #2576, .T. ) ;
#9863=EDGE_LOOP ( 'NONE', ( #5591, #3588, #4466, #4443 ) ) ;
#9885=DIRECTION ( 'NONE',  ( 1.000000000000000000, 0.000000000000000000, -0.000000000000000000 ) ) ;
#9894=FACE_OUTER_BOUND ( 'NONE', #8986, .T. ) ;
#9920=CARTESIAN_POINT ( 'NONE',  ( 51.00000000000000711, 50.00000000000000711, -38.00000000000000000 ) ) ;
#9922=CARTESIAN_POINT ( 'NONE',  ( 51.00000000000000000, -3.499999999999998668, -38.49999999999998579 ) ) ;
#9968=ORIENTED_EDGE ( 'NONE', *, *, #2253, .T. ) ;
#10013=AXIS2_PLACEMENT_3D ( 'NONE', #5292, #6347, #1663 ) ;
#10116=LINE ( 'NONE', #7316, #5598 ) ;
#10144=CARTESIAN_POINT ( 'NONE',  ( 45.00000000000001421, 50.00000000000000711, -38.00000000000000000 ) ) ;
#10151=VECTOR ( 'NONE', #2385, 1000.000000000000000 ) ;
#10181=CARTESIAN_POINT ( 'NONE',  ( 51.00000000000000000, 5.744562646538045492, -38.00000000000000000 ) ) ;
#10195=CARTESIAN_POINT ( 'NONE',  ( 46.00000000000000000, 3.500000000000001332, -45.49999999999998579 ) ) ;
#10198=PRODUCT_DEFINITION_SHAPE ( 'NONE', 'NONE',  #7554 ) ;
#10205=ORIENTED_EDGE ( 'NONE', *, *, #11724, .F. ) ;
#10293=CARTESIAN_POINT ( 'NONE',  ( 45.00000000000001421, 50.00000000000000711, -38.00000000000000000 ) ) ;
#10296=EDGE_LOOP ( 'NONE', ( #378, #3451, #10205, #10472, #5560, #3344 ) ) ;
#10298=ORIENTED_EDGE ( 'NONE', *, *, #2333, .F. ) ;
#10304=CARTESIAN_POINT ( 'NONE',  ( 76.00000000000000000, 46.00000000000001421, -41.99999999999999289 ) ) ;
#10344=CIRCLE ( 'NONE', #2163, 5.000000000000004441 ) ;
#10351=LINE ( 'NONE', #10293, #8210 ) ;
#10390=FACE_BOUND ( 'NONE', #5179, .T. ) ;
#10449=LINE ( 'NONE', #4818, #4900 ) ;
#10450=AXIS2_PLACEMENT_3D ( 'NONE', #7203, #4258, #1509 ) ;
#10472=ORIENTED_EDGE ( 'NONE', *, *, #7216, .F. ) ;
#10474=VERTEX_POINT ( 'NONE', #11304 ) ;
#10482=DIRECTION ( 'NONE',  ( 0.000000000000000000, 0.000000000000000000, 1.000000000000000000 ) ) ;
#10483=CARTESIAN_POINT ( 'NONE',  ( 45.00000000000001421, 7.000000000000004441, -41.99999999999998579 ) ) ;
#10494=CARTESIAN_POINT ( 'NONE',  ( 46.00000000000000000, -3.499999999999998668, -45.49999999999998579 ) ) ;
#10580=EDGE_CURVE ( 'NONE', #8484, #3527, #11543, .T. ) ;
#10596=CIRCLE ( 'NONE', #216, 7.000000000000006217 ) ;
#10599=CIRCLE ( 'NONE', #6616, 5.000000000000004441 ) ;
#10627=VECTOR ( 'NONE', #905, 1000.000000000000000 ) ;
#10669=EDGE_LOOP ( 'NONE', ( #4692, #6726, #5935, #4509, #4226, #8452 ) ) ;
#10704=CARTESIAN_POINT ( 'NONE',  ( 51.00000000000000000, 46.00000000000001421, -46.00000000000000000 ) ) ;
#10715=DIRECTION ( 'NONE',  ( 0.000000000000000000, -0.000000000000000000, 1.000000000000000000 ) ) ;
#10733=ORIENTED_EDGE ( 'NONE', *, *, #7034, .F. ) ;
#10762=EDGE_CURVE ( 'NONE', #811, #1905, #5549, .T. ) ;
#10812=FACE_OUTER_BOUND ( 'NONE', #2603, .T. ) ;
#10820=AXIS2_PLACEMENT_3D ( 'NONE', #6915, #3158, #10715 ) ;
#10886=CARTESIAN_POINT ( 'NONE',  ( 76.00000000000000000, 46.00000000000001421, -46.00000000000000000 ) ) ;
#10888=ORIENTED_EDGE ( 'NONE', *, *, #4335, .T. ) ;
#10929=DIRECTION ( 'NONE',  ( 0.000000000000000000, -1.000000000000000000, 0.000000000000000000 ) ) ;
#10951=AXIS2_PLACEMENT_3D ( 'NONE', #9003, #1176, #7999 ) ;
#10964=CARTESIAN_POINT ( 'NONE',  ( 46.00000000000000000, 1.444447458290426890E-31, -41.99999999999998579 ) ) ;
#10997=CIRCLE ( 'NONE', #1622, 7.000000000000006217 ) ;
#11013=AXIS2_PLACEMENT_3D ( 'NONE', #2006, #11369, #11440 ) ;
#11064=CARTESIAN_POINT ( 'NONE',  ( 65.79898987322334847, 5.744562646538025952, -46.00000000000000000 ) ) ;
#11074=EDGE_LOOP ( 'NONE', ( #3432, #3632 ) ) ;
#11088=ORIENTED_EDGE ( 'NONE', *, *, #1174, .T. ) ;
#11105=DIRECTION ( 'NONE',  ( 0.000000000000000000, 0.000000000000000000, -1.000000000000000000 ) ) ;
#11110=ADVANCED_FACE ( 'NONE', ( #4390 ), #12017, .T. ) ;
#11131=LINE ( 'NONE', #10195, #7432 ) ;
#11135=ADVANCED_FACE ( 'NONE', ( #1652, #10390 ), #4707, .F. ) ;
#11137=FACE_OUTER_BOUND ( 'NONE', #311, .T. ) ;
#11141=AXIS2_PLACEMENT_3D ( 'NONE', #9711, #2130, #5948 ) ;
#11148=VECTOR ( 'NONE', #4234, 1000.000000000000000 ) ;
#11217=LINE ( 'NONE', #12323, #10627 ) ;
#11275=DIRECTION ( 'NONE',  ( -1.000000000000000000, -0.000000000000000000, -0.000000000000000000 ) ) ;
#11296=EDGE_CURVE ( 'NONE', #170, #7890, #10997, .T. ) ;
#11304=CARTESIAN_POINT ( 'NONE',  ( 51.00000000000000000, 3.500000000000001332, -45.49999999999998579 ) ) ;
#11361=LINE ( 'NONE', #6446, #2584 ) ;
#11369=DIRECTION ( 'NONE',  ( 1.000000000000000000, 0.000000000000000000, 0.000000000000000000 ) ) ;
#11384=CARTESIAN_POINT ( 'NONE',  ( 46.00000000000000000, 5.000000000000004441, -41.99999999999998579 ) ) ;
#11394=LINE ( 'NONE', #9410, #361 ) ;
#11396=CARTESIAN_POINT ( 'NONE',  ( 51.00000000000000000, -3.499999999999998668, -45.49999999999998579 ) ) ;
#11407=PRODUCT_CONTEXT ( 'NONE', #5206, 'mechanical' ) ;
#11415=VECTOR ( 'NONE', #2694, 1000.000000000000000 ) ;
#11440=DIRECTION ( 'NONE',  ( 0.000000000000000000, 0.000000000000000000, -1.000000000000000000 ) ) ;
#11457=VECTOR ( 'NONE', #8051, 1000.000000000000000 ) ;
#11469=ORIENTED_EDGE ( 'NONE', *, *, #108, .T. ) ;
#11543=CIRCLE ( 'NONE', #10951, 4.000000000000003553 ) ;
#11646=CARTESIAN_POINT ( 'NONE',  ( 45.00000000000001421, 4.770489558936308102E-18, -41.99999999999998579 ) ) ;
#11652=PLANE ( 'NONE',  #10820 ) ;
#11657=CARTESIAN_POINT ( 'NONE',  ( 51.00000000000000711, 50.00000000000000711, -46.00000000000000000 ) ) ;
#11666=CARTESIAN_POINT ( 'NONE',  ( 0.000000000000000000, 46.00000000000001421, -37.99999999999999289 ) ) ;
#11724=EDGE_CURVE ( 'NONE', #7793, #8701, #8833, .T. ) ;
#11732=SHAPE_REPRESENTATION_RELATIONSHIP ( 'NONE' , 'NONE' ,  #8426, #4358 ) ;
#11734=DIRECTION ( 'NONE',  ( 0.000000000000000000, -1.000000000000000000, 0.000000000000000000 ) ) ;
#11744=DIRECTION ( 'NONE',  ( 1.000000000000000000, 0.000000000000000000, -0.000000000000000000 ) ) ;
#11770=AXIS2_PLACEMENT_3D ( 'NONE', #7365, #7434, #11105 ) ;
#11822=FACE_OUTER_BOUND ( 'NONE', #27, .T. ) ;
#11906=CARTESIAN_POINT ( 'NONE',  ( 65.79898987322334847, -5.000000000000004441, -41.99999999999998579 ) ) ;
#11931=VECTOR ( 'NONE', #3545, 1000.000000000000000 ) ;
#11943=DIRECTION ( 'NONE',  ( -1.000000000000000000, 4.770489558936235687E-18, -6.855277276495154548E-34 ) ) ;
#11956=DIRECTION ( 'NONE',  ( -1.000000000000000000, 0.000000000000000000, -0.000000000000000000 ) ) ;
#11958=LINE ( 'NONE', #3349, #6015 ) ;
#11961=ORIENTED_EDGE ( 'NONE', *, *, #10762, .F. ) ;
#11978=AXIS2_PLACEMENT_3D ( 'NONE', #5186, #4252, #10929 ) ;
#11986=VECTOR ( 'NONE', #7550, 1000.000000000000000 ) ;
#12014=EDGE_LOOP ( 'NONE', ( #7116, #11469, #4351, #10733, #5550 ) ) ;
#12017=CYLINDRICAL_SURFACE ( 'NONE', #3423, 4.000000000000003553 ) ;
#12085=PRODUCT ( 'handle', 'handle', '', ( #11407 ) ) ;
#12095=ORIENTED_EDGE ( 'NONE', *, *, #6325, .T. ) ;
#12124=CARTESIAN_POINT ( 'NONE',  ( 46.00000000000000000, -3.499999999999998668, -38.49999999999998579 ) ) ;
#12126=FACE_OUTER_BOUND ( 'NONE', #8807, .T. ) ;
#12159=DIRECTION ( 'NONE',  ( -0.000000000000000000, -1.000000000000000000, -0.000000000000000000 ) ) ;
#12174=ORIENTED_EDGE ( 'NONE', *, *, #4629, .T. ) ;
#12220=DIRECTION ( 'NONE',  ( 1.000000000000000000, -4.770489558936235687E-18, 6.855277276495153692E-34 ) ) ;
#12259=CARTESIAN_POINT ( 'NONE',  ( 51.00000000000000000, 0.000000000000000000, 0.000000000000000000 ) ) ;
#12296=DIRECTION ( 'NONE',  ( 0.000000000000000000, 1.000000000000000000, 0.000000000000000000 ) ) ;
#12323=CARTESIAN_POINT ( 'NONE',  ( 70.79898987322334847, -3.499999999999998668, -45.49999999999998579 ) ) ;
#12385=COLOUR_RGB('Sky Blue',0.24,0.69,0.87);
#12386=FILL_AREA_STYLE_COLOUR('',#12385);
#12387=FILL_AREA_STYLE('',(#12386));
#12388=SURFACE_STYLE_FILL_AREA(#12387);
#12389=SURFACE_SIDE_STYLE('',(#12388));
#12390=SURFACE_STYLE_USAGE(.BOTH.,#12389);
#12391=PRESENTATION_STYLE_ASSIGNMENT((#12390));
ENDSEC;
END-ISO-10303-21;
